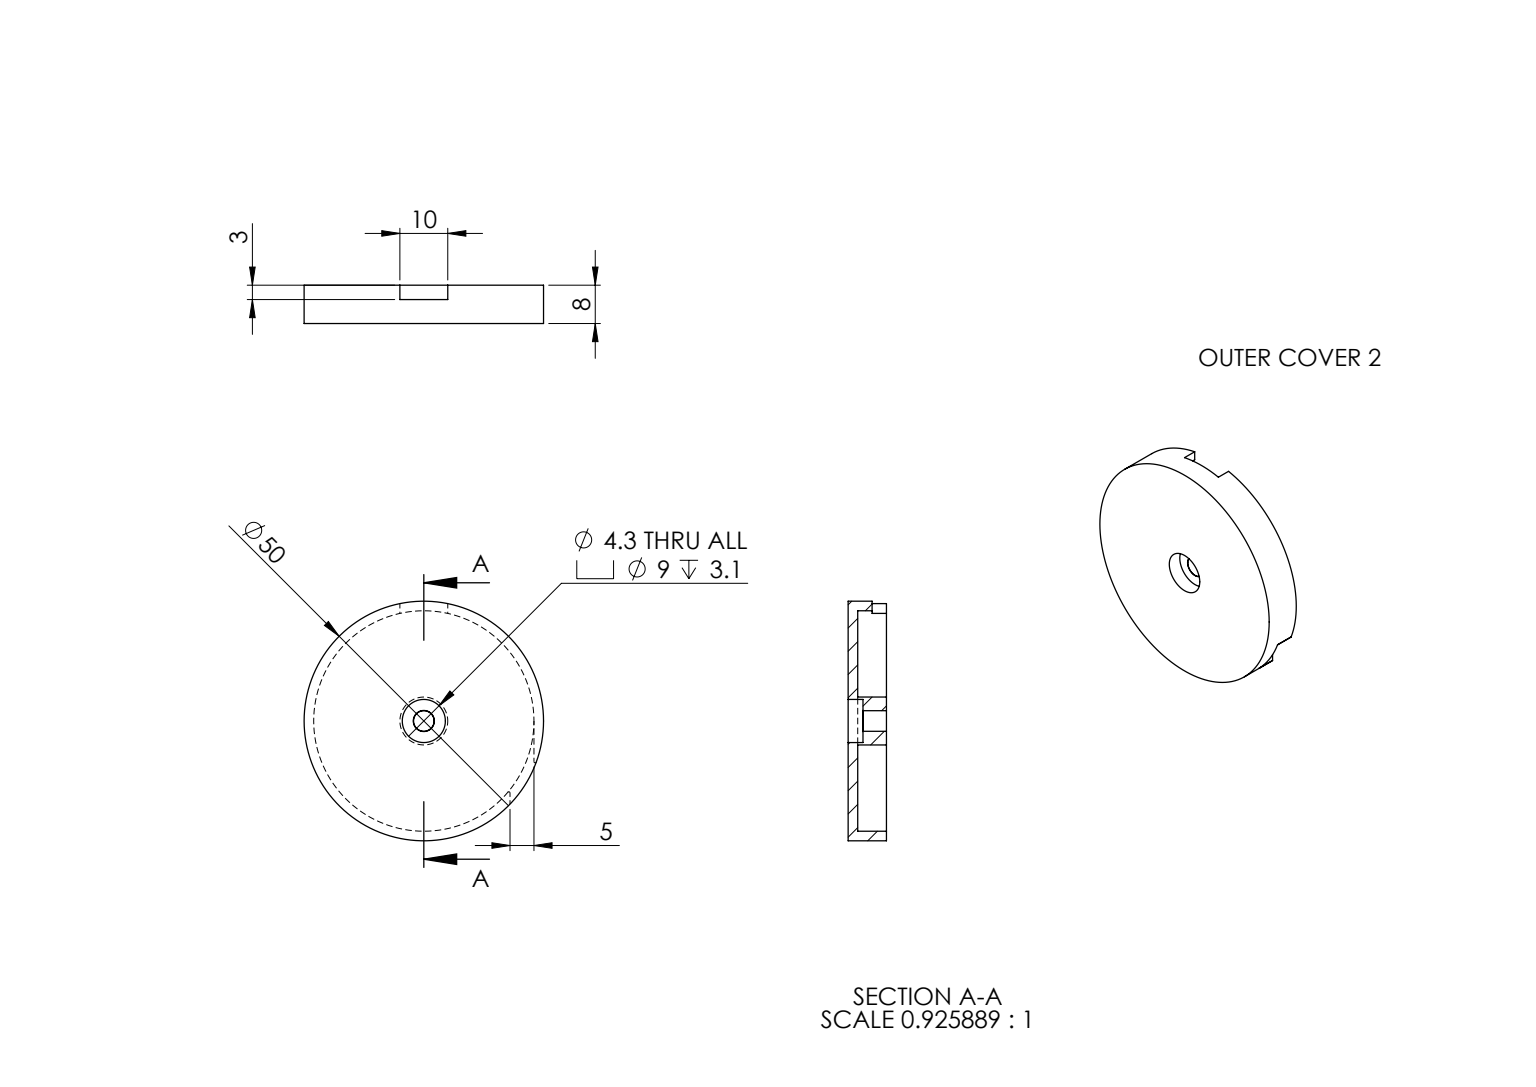
ISO-10303-21;
HEADER;
FILE_DESCRIPTION (('STEP AP214'),
    '1' );
FILE_NAME ('outer cover 2.step',
    '2026-10-23T14:45:25',
    ( '' ),
    ( '' ),
    'SwSTEP 2.0',
    'SolidWorks 2026',
    '' );
FILE_SCHEMA (( 'AUTOMOTIVE_DESIGN' ));
ENDSEC;

DATA;
#3=ORIENTED_EDGE ( 'NONE', *, *, #653, .T. ) ;
#4=EDGE_CURVE ( 'NONE', #1240, #2861, #1350, .T. ) ;
#28=FACE_OUTER_BOUND ( 'NONE', #3065, .T. ) ;
#29=CARTESIAN_POINT ( 'NONE',  ( -25.00000000000000000, 0.000000000000000000, -8.000000000000000000 ) ) ;
#36=VERTEX_POINT ( 'NONE', #2452 ) ;
#37=ORIENTED_EDGE ( 'NONE', *, *, #2017, .F. ) ;
#43=CIRCLE ( 'NONE', #2159, 23.00000000000000000 ) ;
#44=ORIENTED_EDGE ( 'NONE', *, *, #3966, .F. ) ;
#53=DIRECTION ( 'NONE',  ( -0.000000000000000000, -0.000000000000000000, -1.000000000000000000 ) ) ;
#56=CARTESIAN_POINT ( 'NONE',  ( 2.199999999999999289, 0.000000000000000000, -3.300000000000000266 ) ) ;
#58=EDGE_LOOP ( 'NONE', ( #1044, #3800, #158, #292 ) ) ;
#68=AXIS2_PLACEMENT_3D ( 'NONE', #3117, #2273, #3510 ) ;
#82=CARTESIAN_POINT ( 'NONE',  ( -2.149999999999997691, 2.632990618166807263E-16, -8.000000000000000000 ) ) ;
#85=DIRECTION ( 'NONE',  ( 0.000000000000000000, 0.000000000000000000, 1.000000000000000000 ) ) ;
#86=FACE_OUTER_BOUND ( 'NONE', #1906, .T. ) ;
#110=DIRECTION ( 'NONE',  ( -1.000000000000000000, 0.000000000000000000, 0.000000000000000000 ) ) ;
#118=VERTEX_POINT ( 'NONE', #3747 ) ;
#127=CIRCLE ( 'NONE', #405, 23.00000000000000000 ) ;
#130=AXIS2_PLACEMENT_3D ( 'NONE', #3700, #1115, #2554 ) ;
#146=DIRECTION ( 'NONE',  ( 1.000000000000000000, 0.000000000000000000, 0.000000000000000000 ) ) ;
#154=ADVANCED_FACE ( 'NONE', ( #5473 ), #2392, .F. ) ;
#158=ORIENTED_EDGE ( 'NONE', *, *, #190, .T. ) ;
#161=DIRECTION ( 'NONE',  ( -4.364351673553916694E-15, 1.000000000000000000, 0.000000000000000000 ) ) ;
#174=DIRECTION ( 'NONE',  ( 1.000000000000000000, 0.000000000000000000, 0.000000000000000000 ) ) ;
#190=EDGE_CURVE ( 'NONE', #442, #1012, #3278, .T. ) ;
#194=CARTESIAN_POINT ( 'NONE',  ( -25.00000000000000000, 0.000000000000000000, -8.000000000000000000 ) ) ;
#202=CARTESIAN_POINT ( 'NONE',  ( 25.00000000000000000, -3.061616997868383043E-15, -8.000000000000000000 ) ) ;
#204=ORIENTED_EDGE ( 'NONE', *, *, #5079, .F. ) ;
#207=DIRECTION ( 'NONE',  ( 1.000000000000000000, 0.000000000000000000, 0.000000000000000000 ) ) ;
#222=AXIS2_PLACEMENT_3D ( 'NONE', #3534, #53, #4345 ) ;
#225=( NAMED_UNIT ( * ) PLANE_ANGLE_UNIT ( ) SI_UNIT ( $, .RADIAN. ) );
#231=CARTESIAN_POINT ( 'NONE',  ( 0.000000000000000000, 0.000000000000000000, -3.106350832689629637 ) ) ;
#232=ORIENTED_EDGE ( 'NONE', *, *, #2358, .F. ) ;
#233=CIRCLE ( 'NONE', #3913, 2.149999999999997691 ) ;
#235=CARTESIAN_POINT ( 'NONE',  ( 0.000000000000000000, 0.000000000000000000, -8.000000000000000000 ) ) ;
#238=DIRECTION ( 'NONE',  ( -0.000000000000000000, -0.000000000000000000, -1.000000000000000000 ) ) ;
#239=ORIENTED_EDGE ( 'NONE', *, *, #2358, .T. ) ;
#247=VERTEX_POINT ( 'NONE', #3664 ) ;
#254=ORIENTED_EDGE ( 'NONE', *, *, #1540, .F. ) ;
#283=CARTESIAN_POINT ( 'NONE',  ( 0.000000000000000000, 0.000000000000000000, 0.000000000000000000 ) ) ;
#284=CARTESIAN_POINT ( 'NONE',  ( -5.000000000000000000, 0.000000000000000000, -2.000000000000000000 ) ) ;
#285=DIRECTION ( 'NONE',  ( -0.000000000000000000, -0.000000000000000000, 1.000000000000000000 ) ) ;
#287=CARTESIAN_POINT ( 'NONE',  ( 0.000000000000000000, 0.000000000000000000, -8.000000000000000000 ) ) ;
#292=ORIENTED_EDGE ( 'NONE', *, *, #2127, .F. ) ;
#298=PRODUCT_DEFINITION_FORMATION_WITH_SPECIFIED_SOURCE ( 'ANY', '', #4227, .NOT_KNOWN. ) ;
#313=DIRECTION ( 'NONE',  ( 0.000000000000000000, 0.000000000000000000, -1.000000000000000000 ) ) ;
#314=( LENGTH_UNIT ( ) NAMED_UNIT ( * ) SI_UNIT ( .MILLI., .METRE. ) );
#325=ORIENTED_EDGE ( 'NONE', *, *, #4902, .F. ) ;
#334=CIRCLE ( 'NONE', #715, 2.149999999999997691 ) ;
#342=CIRCLE ( 'NONE', #3844, 5.000000000000000000 ) ;
#347=CARTESIAN_POINT ( 'NONE',  ( 2.149999999999997691, 0.000000000000000000, -8.000000000000000000 ) ) ;
#352=EDGE_CURVE ( 'NONE', #3586, #36, #4839, .T. ) ;
#353=CARTESIAN_POINT ( 'NONE',  ( 23.00000000000000000, -2.816687638038912352E-15, -8.000000000000000000 ) ) ;
#354=VERTEX_POINT ( 'NONE', #2939 ) ;
#355=DIRECTION ( 'NONE',  ( -0.000000000000000000, -0.000000000000000000, 1.000000000000000000 ) ) ;
#370=FACE_OUTER_BOUND ( 'NONE', #4591, .T. ) ;
#379=ORIENTED_EDGE ( 'NONE', *, *, #1622, .F. ) ;
#387=ORIENTED_EDGE ( 'NONE', *, *, #3947, .T. ) ;
#401=CIRCLE ( 'NONE', #1231, 25.00000000000000000 ) ;
#403=VERTEX_POINT ( 'NONE', #4665 ) ;
#405=AXIS2_PLACEMENT_3D ( 'NONE', #490, #1846, #5415 ) ;
#410=CARTESIAN_POINT ( 'NONE',  ( 17.99999999999999289, -15.01665741768121443, -4.000000000000000000 ) ) ;
#412=EDGE_CURVE ( 'NONE', #4755, #1305, #3551, .T. ) ;
#418=DIRECTION ( 'NONE',  ( -0.000000000000000000, -0.000000000000000000, 1.000000000000000000 ) ) ;
#429=EDGE_CURVE ( 'NONE', #1326, #5392, #2179, .T. ) ;
#432=DIRECTION ( 'NONE',  ( 1.000000000000000000, 4.364351673553916694E-15, 0.000000000000000000 ) ) ;
#434=PLANE ( 'NONE',  #1688 ) ;
#437=LINE ( 'NONE', #5272, #4474 ) ;
#442=VERTEX_POINT ( 'NONE', #2044 ) ;
#447=DIRECTION ( 'NONE',  ( 1.000000000000000000, 0.000000000000000000, 0.000000000000000000 ) ) ;
#449=ORIENTED_EDGE ( 'NONE', *, *, #2127, .T. ) ;
#463=CARTESIAN_POINT ( 'NONE',  ( -5.000000000000076383, 22.44994432064363110, -8.000000000000000000 ) ) ;
#480=CARTESIAN_POINT ( 'NONE',  ( 5.000000000000000000, -6.123233995736766282E-16, -8.000000000000000000 ) ) ;
#485=ORIENTED_EDGE ( 'NONE', *, *, #2804, .F. ) ;
#488=ADVANCED_FACE ( 'NONE', ( #1241, #3003 ), #4748, .T. ) ;
#490=CARTESIAN_POINT ( 'NONE',  ( 0.000000000000000000, 0.000000000000000000, -4.000000000000000000 ) ) ;
#505=VECTOR ( 'NONE', #782, 1000.000000000000000 ) ;
#519=CARTESIAN_POINT ( 'NONE',  ( 0.000000000000000000, 0.000000000000000000, 0.000000000000000000 ) ) ;
#521=DIRECTION ( 'NONE',  ( 1.000000000000000000, 0.000000000000000000, 0.000000000000000000 ) ) ;
#529=VECTOR ( 'NONE', #2822, 1000.000000000000000 ) ;
#530=EDGE_CURVE ( 'NONE', #964, #1719, #3971, .T. ) ;
#533=VECTOR ( 'NONE', #2608, 1000.000000000000000 ) ;
#541=CARTESIAN_POINT ( 'NONE',  ( 4.999999999999914735, 24.49489742783179835, -8.000000000000000000 ) ) ;
#545=DIRECTION ( 'NONE',  ( -0.000000000000000000, -0.000000000000000000, 1.000000000000000000 ) ) ;
#547=CARTESIAN_POINT ( 'NONE',  ( 0.000000000000000000, 0.000000000000000000, -8.000000000000000000 ) ) ;
#559=EDGE_CURVE ( 'NONE', #5009, #2746, #334, .T. ) ;
#595=AXIS2_PLACEMENT_3D ( 'NONE', #235, #4212, #754 ) ;
#617=CARTESIAN_POINT ( 'NONE',  ( 0.000000000000000000, 0.000000000000000000, -2.000000000000000000 ) ) ;
#629=LINE ( 'NONE', #194, #3082 ) ;
#630=SURFACE_STYLE_FILL_AREA ( #1056 ) ;
#637=FACE_OUTER_BOUND ( 'NONE', #4150, .T. ) ;
#639=DIRECTION ( 'NONE',  ( 0.000000000000000000, 0.000000000000000000, -1.000000000000000000 ) ) ;
#640=ORIENTED_EDGE ( 'NONE', *, *, #4759, .T. ) ;
#653=EDGE_CURVE ( 'NONE', #2224, #1028, #888, .T. ) ;
#655=ORIENTED_EDGE ( 'NONE', *, *, #4575, .F. ) ;
#658=( LENGTH_UNIT ( ) NAMED_UNIT ( * ) SI_UNIT ( .MILLI., .METRE. ) );
#679=EDGE_CURVE ( 'NONE', #5392, #4001, #437, .T. ) ;
#684=PRODUCT_DEFINITION_SHAPE ( 'NONE', 'NONE',  #4858 ) ;
#685=CIRCLE ( 'NONE', #222, 0.2500000000000002220 ) ;
#697=DIRECTION ( 'NONE',  ( 1.000000000000000000, 0.000000000000000000, 0.000000000000000000 ) ) ;
#706=AXIS2_PLACEMENT_3D ( 'NONE', #231, #639, #3316 ) ;
#715=AXIS2_PLACEMENT_3D ( 'NONE', #547, #1756, #4837 ) ;
#726=VERTEX_POINT ( 'NONE', #4122 ) ;
#734=ORIENTED_EDGE ( 'NONE', *, *, #788, .F. ) ;
#749=DIRECTION ( 'NONE',  ( -1.000000000000000000, 0.000000000000000000, -0.000000000000000000 ) ) ;
#750=FACE_OUTER_BOUND ( 'NONE', #5246, .T. ) ;
#751=ORIENTED_EDGE ( 'NONE', *, *, #1982, .T. ) ;
#754=DIRECTION ( 'NONE',  ( 1.000000000000000000, 0.000000000000000000, 0.000000000000000000 ) ) ;
#777=AXIS2_PLACEMENT_3D ( 'NONE', #4406, #5273, #4868 ) ;
#782=DIRECTION ( 'NONE',  ( 0.000000000000000000, 0.000000000000000000, -1.000000000000000000 ) ) ;
#788=EDGE_CURVE ( 'NONE', #1305, #1719, #3740, .T. ) ;
#789=ORIENTED_EDGE ( 'NONE', *, *, #2529, .F. ) ;
#804=CARTESIAN_POINT ( 'NONE',  ( 0.000000000000000000, 0.000000000000000000, -8.000000000000000000 ) ) ;
#805=AXIS2_PLACEMENT_3D ( 'NONE', #2161, #2766, #5035 ) ;
#808=VECTOR ( 'NONE', #3588, 1000.000000000000000 ) ;
#810=DIRECTION ( 'NONE',  ( -0.000000000000000000, -0.000000000000000000, 1.000000000000000000 ) ) ;
#818=ORIENTED_EDGE ( 'NONE', *, *, #1286, .T. ) ;
#836=CARTESIAN_POINT ( 'NONE',  ( 23.00000000000000000, -2.168404344971008868E-16, -4.000000000000000000 ) ) ;
#840=LINE ( 'NONE', #2596, #1777 ) ;
#848=MECHANICAL_DESIGN_GEOMETRIC_PRESENTATION_REPRESENTATION('',(#4251),#2780);
#860=CARTESIAN_POINT ( 'NONE',  ( 23.00000000000000000, -2.168404344971008868E-16, -8.000000000000000000 ) ) ;
#862=CARTESIAN_POINT ( 'NONE',  ( 2.149999999999998579, 0.000000000000000000, 0.000000000000000000 ) ) ;
#864=DIRECTION ( 'NONE',  ( 1.000000000000000000, 0.000000000000000000, 0.000000000000000000 ) ) ;
#867=AXIS2_PLACEMENT_3D ( 'NONE', #4433, #2247, #5330 ) ;
#869=DIRECTION ( 'NONE',  ( -3.540989467475305966E-16, -1.000000000000000000, -0.000000000000000000 ) ) ;
#872=ORIENTED_EDGE ( 'NONE', *, *, #3851, .T. ) ;
#873=CIRCLE ( 'NONE', #595, 25.00000000000000000 ) ;
#878=FACE_OUTER_BOUND ( 'NONE', #5457, .T. ) ;
#882=AXIS2_PLACEMENT_3D ( 'NONE', #2501, #810, #3833 ) ;
#888=CIRCLE ( 'NONE', #3930, 4.500000000000000000 ) ;
#889=DIRECTION ( 'NONE',  ( -3.540989467475305966E-16, -1.000000000000000000, -0.000000000000000000 ) ) ;
#893=CARTESIAN_POINT ( 'NONE',  ( -23.00000000000000000, 0.000000000000000000, -8.000000000000000000 ) ) ;
#894=APPLICATION_CONTEXT ( 'automotive_design' ) ;
#896=DIRECTION ( 'NONE',  ( -4.364351673553916694E-15, 1.000000000000000000, 0.000000000000000000 ) ) ;
#901=ORIENTED_EDGE ( 'NONE', *, *, #5146, .T. ) ;
#920=CARTESIAN_POINT ( 'NONE',  ( 0.000000000000000000, 0.000000000000000000, -5.000000000000000000 ) ) ;
#921=DIRECTION ( 'NONE',  ( 1.000000000000000000, 0.000000000000000000, 0.000000000000000000 ) ) ;
#922=ORIENTED_EDGE ( 'NONE', *, *, #4867, .T. ) ;
#924=FACE_OUTER_BOUND ( 'NONE', #1877, .T. ) ;
#926=DIRECTION ( 'NONE',  ( -0.000000000000000000, -0.000000000000000000, 1.000000000000000000 ) ) ;
#929=ORIENTED_EDGE ( 'NONE', *, *, #5527, .F. ) ;
#948=DIRECTION ( 'NONE',  ( 0.000000000000000000, -1.000000000000000000, 0.000000000000000000 ) ) ;
#953=SHAPE_REPRESENTATION ( 'outer cover 2', ( #1336 ), #1859 ) ;
#964=VERTEX_POINT ( 'NONE', #4986 ) ;
#968=VECTOR ( 'NONE', #1615, 1000.000000000000000 ) ;
#971=ORIENTED_EDGE ( 'NONE', *, *, #1622, .T. ) ;
#974=DIRECTION ( 'NONE',  ( 0.000000000000000000, 0.000000000000000000, -1.000000000000000000 ) ) ;
#976=LINE ( 'NONE', #3168, #5554 ) ;
#978=PLANE ( 'NONE',  #1040 ) ;
#1009=FACE_BOUND ( 'NONE', #1425, .T. ) ;
#1011=CARTESIAN_POINT ( 'NONE',  ( 0.000000000000000000, 0.000000000000000000, -8.000000000000000000 ) ) ;
#1012=VERTEX_POINT ( 'NONE', #4674 ) ;
#1013=DIRECTION ( 'NONE',  ( -3.540989467475305966E-16, -1.000000000000000000, -0.000000000000000000 ) ) ;
#1028=VERTEX_POINT ( 'NONE', #2977 ) ;
#1033=DIRECTION ( 'NONE',  ( -3.540989467475305966E-16, -1.000000000000000000, -0.000000000000000000 ) ) ;
#1040=AXIS2_PLACEMENT_3D ( 'NONE', #2620, #432, #2736 ) ;
#1044=ORIENTED_EDGE ( 'NONE', *, *, #653, .F. ) ;
#1054=AXIS2_PLACEMENT_3D ( 'NONE', #2328, #1955, #1472 ) ;
#1056=FILL_AREA_STYLE ('',( #3198 ) ) ;
#1080=AXIS2_PLACEMENT_3D ( 'NONE', #5289, #3105, #5452 ) ;
#1090=DIRECTION ( 'NONE',  ( 1.000000000000000000, 0.000000000000000000, 0.000000000000000000 ) ) ;
#1106=ORIENTED_EDGE ( 'NONE', *, *, #4480, .T. ) ;
#1112=ORIENTED_EDGE ( 'NONE', *, *, #3851, .F. ) ;
#1115=DIRECTION ( 'NONE',  ( -0.000000000000000000, -0.000000000000000000, 1.000000000000000000 ) ) ;
#1121=FACE_OUTER_BOUND ( 'NONE', #1958, .T. ) ;
#1130=ORIENTED_EDGE ( 'NONE', *, *, #4867, .F. ) ;
#1143=FACE_OUTER_BOUND ( 'NONE', #1789, .T. ) ;
#1146=ORIENTED_EDGE ( 'NONE', *, *, #3983, .F. ) ;
#1150=CYLINDRICAL_SURFACE ( 'NONE', #4567, 25.00000000000000000 ) ;
#1154=CYLINDRICAL_SURFACE ( 'NONE', #882, 5.000000000000000000 ) ;
#1155=ORIENTED_EDGE ( 'NONE', *, *, #4164, .T. ) ;
#1165=FACE_OUTER_BOUND ( 'NONE', #5587, .T. ) ;
#1188=DIRECTION ( 'NONE',  ( -0.000000000000000000, -0.000000000000000000, -1.000000000000000000 ) ) ;
#1189=CARTESIAN_POINT ( 'NONE',  ( -4.500000000000000000, 5.510910596163088569E-16, -3.100000000000000533 ) ) ;
#1215=ORIENTED_EDGE ( 'NONE', *, *, #3973, .F. ) ;
#1221=ORIENTED_EDGE ( 'NONE', *, *, #3980, .F. ) ;
#1231=AXIS2_PLACEMENT_3D ( 'NONE', #5535, #4721, #2082 ) ;
#1240=VERTEX_POINT ( 'NONE', #3493 ) ;
#1241=FACE_BOUND ( 'NONE', #2539, .T. ) ;
#1243=AXIS2_PLACEMENT_3D ( 'NONE', #5613, #2971, #4485 ) ;
#1251=VERTEX_POINT ( 'NONE', #893 ) ;
#1256=CIRCLE ( 'NONE', #1987, 0.2000000000000000944 ) ;
#1271=LINE ( 'NONE', #836, #5014 ) ;
#1274=EDGE_CURVE ( 'NONE', #2861, #1240, #2182, .T. ) ;
#1275=DIRECTION ( 'NONE',  ( -1.000000000000000000, 0.000000000000000000, 0.000000000000000000 ) ) ;
#1280=CARTESIAN_POINT ( 'NONE',  ( -5.000000000000076383, 22.44994432064363110, -8.000000000000000000 ) ) ;
#1283=VERTEX_POINT ( 'NONE', #5298 ) ;
#1286=EDGE_CURVE ( 'NONE', #4444, #1251, #4750, .T. ) ;
#1300=LINE ( 'NONE', #5154, #4925 ) ;
#1303=CARTESIAN_POINT ( 'NONE',  ( 0.000000000000000000, 0.000000000000000000, -3.100000000000000533 ) ) ;
#1305=VERTEX_POINT ( 'NONE', #29 ) ;
#1326=VERTEX_POINT ( 'NONE', #2652 ) ;
#1335=DIRECTION ( 'NONE',  ( 1.000000000000000000, 0.000000000000000000, 0.000000000000000000 ) ) ;
#1336=AXIS2_PLACEMENT_3D ( 'NONE', #283, #2997, #5213 ) ;
#1339=VECTOR ( 'NONE', #4158, 1000.000000000000000 ) ;
#1350=CIRCLE ( 'NONE', #5207, 25.00000000000000000 ) ;
#1359=FACE_OUTER_BOUND ( 'NONE', #58, .T. ) ;
#1363=AXIS2_PLACEMENT_3D ( 'NONE', #3047, #2232, #4792 ) ;
#1368=EDGE_CURVE ( 'NONE', #4473, #118, #5491, .T. ) ;
#1385=DIRECTION ( 'NONE',  ( -0.000000000000000000, -0.000000000000000000, 1.000000000000000000 ) ) ;
#1388=CARTESIAN_POINT ( 'NONE',  ( 17.99999999999999289, -17.34935157289748631, -8.000000000000000000 ) ) ;
#1406=DIRECTION ( 'NONE',  ( -0.000000000000000000, -0.000000000000000000, 1.000000000000000000 ) ) ;
#1410=CARTESIAN_POINT ( 'NONE',  ( -2.149999999999998579, 2.632990618166807756E-16, 0.000000000000000000 ) ) ;
#1413=AXIS2_PLACEMENT_3D ( 'NONE', #3624, #3999, #2272 ) ;
#1416=ORIENTED_EDGE ( 'NONE', *, *, #5052, .T. ) ;
#1423=EDGE_CURVE ( 'NONE', #5009, #4159, #3539, .T. ) ;
#1425=EDGE_LOOP ( 'NONE', ( #1744, #4928 ) ) ;
#1429=CIRCLE ( 'NONE', #5468, 4.500000000000000000 ) ;
#1433=VECTOR ( 'NONE', #1967, 1000.000000000000000 ) ;
#1435=ADVANCED_FACE ( 'NONE', ( #1359 ), #4864, .F. ) ;
#1436=CARTESIAN_POINT ( 'NONE',  ( 0.000000000000000000, 0.000000000000000000, -5.000000000000000000 ) ) ;
#1438=AXIS2_PLACEMENT_3D ( 'NONE', #56, #948, #4057 ) ;
#1440=EDGE_LOOP ( 'NONE', ( #3729, #3554, #4497, #1761, #1130, #655 ) ) ;
#1442=CARTESIAN_POINT ( 'NONE',  ( -23.00000000000000000, 0.000000000000000000, -8.000000000000000000 ) ) ;
#1467=ADVANCED_FACE ( 'NONE', ( #86 ), #1841, .F. ) ;
#1472=DIRECTION ( 'NONE',  ( 1.000000000000000000, 0.000000000000000000, 0.000000000000000000 ) ) ;
#1479=LINE ( 'NONE', #3236, #1433 ) ;
#1507=CARTESIAN_POINT ( 'NONE',  ( -5.000000000000000000, 4.999999999999978684, -5.000000000000000000 ) ) ;
#1509=CIRCLE ( 'NONE', #777, 23.00000000000000000 ) ;
#1518=PRESENTATION_STYLE_ASSIGNMENT (( #5461 ) ) ;
#1525=CARTESIAN_POINT ( 'NONE',  ( 0.000000000000000000, 0.000000000000000000, -8.000000000000000000 ) ) ;
#1528=AXIS2_PLACEMENT_3D ( 'NONE', #2132, #2912, #2480 ) ;
#1531=ORIENTED_EDGE ( 'NONE', *, *, #4413, .F. ) ;
#1540=EDGE_CURVE ( 'NONE', #3849, #354, #342, .T. ) ;
#1541=ORIENTED_EDGE ( 'NONE', *, *, #3983, .T. ) ;
#1554=( LENGTH_UNIT ( ) NAMED_UNIT ( * ) SI_UNIT ( .MILLI., .METRE. ) );
#1556=VERTEX_POINT ( 'NONE', #1869 ) ;
#1563=DIRECTION ( 'NONE',  ( 1.000000000000000000, 0.000000000000000000, 0.000000000000000000 ) ) ;
#1577=FACE_OUTER_BOUND ( 'NONE', #5516, .T. ) ;
#1579=ORIENTED_EDGE ( 'NONE', *, *, #2603, .F. ) ;
#1592=ORIENTED_EDGE ( 'NONE', *, *, #530, .F. ) ;
#1604=AXIS2_PLACEMENT_3D ( 'NONE', #1750, #3479, #3652 ) ;
#1605=CYLINDRICAL_SURFACE ( 'NONE', #2246, 25.00000000000000000 ) ;
#1615=DIRECTION ( 'NONE',  ( -0.000000000000000000, -0.000000000000000000, 1.000000000000000000 ) ) ;
#1622=EDGE_CURVE ( 'NONE', #1251, #1556, #1925, .T. ) ;
#1631=AXIS2_PLACEMENT_3D ( 'NONE', #2021, #3289, #1563 ) ;
#1647=ORIENTED_EDGE ( 'NONE', *, *, #1995, .F. ) ;
#1651=ADVANCED_BREP_SHAPE_REPRESENTATION ( '', ( #2595, #1336 ), #1859 ) ;
#1654=DIRECTION ( 'NONE',  ( -0.000000000000000000, -0.000000000000000000, 1.000000000000000000 ) ) ;
#1671=CARTESIAN_POINT ( 'NONE',  ( -5.000000000000000000, 0.000000000000000000, -8.000000000000000000 ) ) ;
#1679=EDGE_LOOP ( 'NONE', ( #3362, #5619, #5333, #2493 ) ) ;
#1688=AXIS2_PLACEMENT_3D ( 'NONE', #2651, #85, #4800 ) ;
#1696=VECTOR ( 'NONE', #1406, 1000.000000000000000 ) ;
#1706=DIRECTION ( 'NONE',  ( 0.000000000000000000, 0.000000000000000000, -1.000000000000000000 ) ) ;
#1707=AXIS2_PLACEMENT_3D ( 'NONE', #3491, #355, #2109 ) ;
#1719=VERTEX_POINT ( 'NONE', #3282 ) ;
#1721=PLANE ( 'NONE',  #5033 ) ;
#1731=LINE ( 'NONE', #2999, #2262 ) ;
#1744=ORIENTED_EDGE ( 'NONE', *, *, #1866, .F. ) ;
#1745=DIRECTION ( 'NONE',  ( 1.000000000000000000, 4.364351673553916694E-15, 0.000000000000000000 ) ) ;
#1750=CARTESIAN_POINT ( 'NONE',  ( 0.000000000000000000, 0.000000000000000000, 0.000000000000000000 ) ) ;
#1754=DIRECTION ( 'NONE',  ( -0.000000000000000000, -0.000000000000000000, 1.000000000000000000 ) ) ;
#1756=DIRECTION ( 'NONE',  ( -0.000000000000000000, -0.000000000000000000, 1.000000000000000000 ) ) ;
#1761=ORIENTED_EDGE ( 'NONE', *, *, #4480, .F. ) ;
#1769=ORIENTED_EDGE ( 'NONE', *, *, #3650, .T. ) ;
#1771=LINE ( 'NONE', #3527, #533 ) ;
#1774=SHAPE_DEFINITION_REPRESENTATION ( #684, #953 ) ;
#1777=VECTOR ( 'NONE', #869, 1000.000000000000000 ) ;
#1781=CARTESIAN_POINT ( 'NONE',  ( 23.24999999999999645, -8.485281374238580199, -8.000000000000000000 ) ) ;
#1789=EDGE_LOOP ( 'NONE', ( #922, #4542, #3410, #4328 ) ) ;
#1790=AXIS2_PLACEMENT_3D ( 'NONE', #1436, #3194, #4944 ) ;
#1795=ADVANCED_FACE ( 'NONE', ( #3794 ), #1150, .T. ) ;
#1810=FACE_OUTER_BOUND ( 'NONE', #2083, .T. ) ;
#1812=CIRCLE ( 'NONE', #2462, 4.500000000000000888 ) ;
#1813=CYLINDRICAL_SURFACE ( 'NONE', #1413, 23.00000000000000000 ) ;
#1823=CARTESIAN_POINT ( 'NONE',  ( 0.000000000000000000, 0.000000000000000000, 0.000000000000000000 ) ) ;
#1833=PRODUCT_CONTEXT ( 'NONE', #1998, 'mechanical' ) ;
#1837=CARTESIAN_POINT ( 'NONE',  ( 22.99999999999999645, -8.485281374238580199, -8.000000000000000000 ) ) ;
#1841=CYLINDRICAL_SURFACE ( 'NONE', #805, 23.00000000000000000 ) ;
#1846=DIRECTION ( 'NONE',  ( -0.000000000000000000, -0.000000000000000000, -1.000000000000000000 ) ) ;
#1855=ORIENTED_EDGE ( 'NONE', *, *, #2354, .F. ) ;
#1857=CARTESIAN_POINT ( 'NONE',  ( -5.000000000000000000, 0.000000000000000000, -8.000000000000000000 ) ) ;
#1859=( GEOMETRIC_REPRESENTATION_CONTEXT ( 3 ) GLOBAL_UNCERTAINTY_ASSIGNED_CONTEXT ( ( #2115 ) ) GLOBAL_UNIT_ASSIGNED_CONTEXT ( ( #658, #225, #5030 ) ) REPRESENTATION_CONTEXT ( 'NONE', 'WORKASPACE' ) );
#1866=EDGE_CURVE ( 'NONE', #1012, #442, #1812, .T. ) ;
#1868=DIRECTION ( 'NONE',  ( -0.000000000000000000, -0.000000000000000000, -1.000000000000000000 ) ) ;
#1869=CARTESIAN_POINT ( 'NONE',  ( -23.00000000000000000, 0.000000000000000000, -2.000000000000000000 ) ) ;
#1870=VECTOR ( 'NONE', #3544, 1000.000000000000000 ) ;
#1874=FACE_OUTER_BOUND ( 'NONE', #2278, .T. ) ;
#1875=DIRECTION ( 'NONE',  ( -1.000000000000000000, 0.000000000000000000, 0.000000000000000000 ) ) ;
#1877=EDGE_LOOP ( 'NONE', ( #2752, #4571, #2770, #44 ) ) ;
#1883=AXIS2_PLACEMENT_3D ( 'NONE', #3941, #2586, #4886 ) ;
#1906=EDGE_LOOP ( 'NONE', ( #4564, #3540, #1647, #2028, #971, #2722 ) ) ;
#1925=LINE ( 'NONE', #1442, #529 ) ;
#1935=ADVANCED_FACE ( 'NONE', ( #4419 ), #1721, .F. ) ;
#1947=DIRECTION ( 'NONE',  ( -0.000000000000000000, -0.000000000000000000, 1.000000000000000000 ) ) ;
#1955=DIRECTION ( 'NONE',  ( -0.000000000000000000, -0.000000000000000000, 1.000000000000000000 ) ) ;
#1958=EDGE_LOOP ( 'NONE', ( #4056, #387, #2428, #1215 ) ) ;
#1960=LINE ( 'NONE', #541, #505 ) ;
#1967=DIRECTION ( 'NONE',  ( -0.000000000000000000, -0.000000000000000000, 1.000000000000000000 ) ) ;
#1979=CARTESIAN_POINT ( 'NONE',  ( 17.74999999999999289, -15.01665741768121443, -8.000000000000000000 ) ) ;
#1981=VECTOR ( 'NONE', #3298, 1000.000000000000000 ) ;
#1982=EDGE_CURVE ( 'NONE', #118, #4473, #4572, .T. ) ;
#1987=AXIS2_PLACEMENT_3D ( 'NONE', #4347, #4489, #3509 ) ;
#1989=AXIS2_PLACEMENT_3D ( 'NONE', #2163, #1188, #1275 ) ;
#1995=EDGE_CURVE ( 'NONE', #5065, #4764, #1771, .T. ) ;
#1998=APPLICATION_CONTEXT ( 'automotive_design' ) ;
#2001=CARTESIAN_POINT ( 'NONE',  ( 4.999999999999923617, 22.44994432064366308, -5.000000000000000000 ) ) ;
#2013=ORIENTED_EDGE ( 'NONE', *, *, #4, .T. ) ;
#2017=EDGE_CURVE ( 'NONE', #2140, #4992, #4026, .T. ) ;
#2021=CARTESIAN_POINT ( 'NONE',  ( 0.000000000000000000, 0.000000000000000000, 0.000000000000000000 ) ) ;
#2028=ORIENTED_EDGE ( 'NONE', *, *, #5146, .F. ) ;
#2032=EDGE_CURVE ( 'NONE', #403, #5536, #4075, .T. ) ;
#2043=ORIENTED_EDGE ( 'NONE', *, *, #530, .T. ) ;
#2044=CARTESIAN_POINT ( 'NONE',  ( -4.500000000000000888, 5.510910596163089556E-16, 0.000000000000000000 ) ) ;
#2050=ORIENTED_EDGE ( 'NONE', *, *, #2603, .T. ) ;
#2058=AXIS2_PLACEMENT_3D ( 'NONE', #2680, #4895, #1033 ) ;
#2068=AXIS2_PLACEMENT_3D ( 'NONE', #3708, #4178, #697 ) ;
#2078=DIRECTION ( 'NONE',  ( -0.000000000000000000, -0.000000000000000000, 1.000000000000000000 ) ) ;
#2082=DIRECTION ( 'NONE',  ( 1.000000000000000000, 0.000000000000000000, 0.000000000000000000 ) ) ;
#2083=EDGE_LOOP ( 'NONE', ( #2944, #734, #5367, #4678, #818, #901, #1855 ) ) ;
#2105=LINE ( 'NONE', #1837, #3908 ) ;
#2107=DIRECTION ( 'NONE',  ( 1.000000000000000000, 0.000000000000000000, 0.000000000000000000 ) ) ;
#2109=DIRECTION ( 'NONE',  ( 1.000000000000000000, 0.000000000000000000, 0.000000000000000000 ) ) ;
#2115=UNCERTAINTY_MEASURE_WITH_UNIT (LENGTH_MEASURE( 1.000000000000000082E-05 ), #658, 'distance_accuracy_value', 'NONE');
#2119=EDGE_LOOP ( 'NONE', ( #2510, #239, #3392, #1112 ) ) ;
#2125=DIRECTION ( 'NONE',  ( -1.000000000000000000, 0.000000000000000000, 0.000000000000000000 ) ) ;
#2127=EDGE_CURVE ( 'NONE', #1028, #1012, #2314, .T. ) ;
#2132=CARTESIAN_POINT ( 'NONE',  ( 0.000000000000000000, 0.000000000000000000, -8.000000000000000000 ) ) ;
#2140=VERTEX_POINT ( 'NONE', #1857 ) ;
#2159=AXIS2_PLACEMENT_3D ( 'NONE', #2408, #4540, #3197 ) ;
#2161=CARTESIAN_POINT ( 'NONE',  ( 0.000000000000000000, 0.000000000000000000, -8.000000000000000000 ) ) ;
#2163=CARTESIAN_POINT ( 'NONE',  ( 23.24999999999999645, -8.485281374238580199, -4.000000000000000000 ) ) ;
#2168=VERTEX_POINT ( 'NONE', #4938 ) ;
#2169=CARTESIAN_POINT ( 'NONE',  ( 0.000000000000000000, 0.000000000000000000, -8.000000000000000000 ) ) ;
#2175=AXIS2_PLACEMENT_3D ( 'NONE', #920, #1868, #110 ) ;
#2179=CIRCLE ( 'NONE', #2729, 23.00000000000000000 ) ;
#2182=CIRCLE ( 'NONE', #2915, 25.00000000000000000 ) ;
#2184=ORIENTED_EDGE ( 'NONE', *, *, #4565, .F. ) ;
#2187=PLANE ( 'NONE',  #1883 ) ;
#2193=DIRECTION ( 'NONE',  ( 0.000000000000000000, 0.000000000000000000, -1.000000000000000000 ) ) ;
#2198=ORIENTED_EDGE ( 'NONE', *, *, #3915, .F. ) ;
#2204=DIRECTION ( 'NONE',  ( 0.000000000000000000, 0.000000000000000000, -1.000000000000000000 ) ) ;
#2219=EDGE_LOOP ( 'NONE', ( #4311, #3579, #2918, #5649 ) ) ;
#2222=DIRECTION ( 'NONE',  ( -0.000000000000000000, -0.000000000000000000, 1.000000000000000000 ) ) ;
#2224=VERTEX_POINT ( 'NONE', #1189 ) ;
#2228=EDGE_CURVE ( 'NONE', #247, #4608, #873, .T. ) ;
#2232=DIRECTION ( 'NONE',  ( -0.000000000000000000, -0.000000000000000000, 1.000000000000000000 ) ) ;
#2242=LINE ( 'NONE', #862, #5205 ) ;
#2246=AXIS2_PLACEMENT_3D ( 'NONE', #3764, #4228, #4682 ) ;
#2247=DIRECTION ( 'NONE',  ( -0.000000000000000000, -0.000000000000000000, 1.000000000000000000 ) ) ;
#2248=PLANE ( 'NONE',  #2058 ) ;
#2255=AXIS2_PLACEMENT_3D ( 'NONE', #617, #5537, #3692 ) ;
#2262=VECTOR ( 'NONE', #313, 1000.000000000000000 ) ;
#2269=LINE ( 'NONE', #4453, #2615 ) ;
#2272=DIRECTION ( 'NONE',  ( -1.000000000000000000, 0.000000000000000000, 0.000000000000000000 ) ) ;
#2273=DIRECTION ( 'NONE',  ( -0.000000000000000000, -0.000000000000000000, 1.000000000000000000 ) ) ;
#2278=EDGE_LOOP ( 'NONE', ( #2198, #3250, #5233, #4878 ) ) ;
#2294=( NAMED_UNIT ( * ) SI_UNIT ( $, .STERADIAN. ) SOLID_ANGLE_UNIT ( ) );
#2298=DIRECTION ( 'NONE',  ( -0.000000000000000000, -0.000000000000000000, 1.000000000000000000 ) ) ;
#2300=EDGE_CURVE ( 'NONE', #1028, #2224, #1429, .T. ) ;
#2314=LINE ( 'NONE', #3695, #808 ) ;
#2328=CARTESIAN_POINT ( 'NONE',  ( 0.000000000000000000, 0.000000000000000000, -3.300000000000000266 ) ) ;
#2354=EDGE_CURVE ( 'NONE', #4137, #5065, #5382, .T. ) ;
#2358=EDGE_CURVE ( 'NONE', #2168, #4001, #1960, .T. ) ;
#2366=AXIS2_PLACEMENT_3D ( 'NONE', #519, #2677, #921 ) ;
#2371=CARTESIAN_POINT ( 'NONE',  ( 5.000000000000000000, 5.000000000000022204, -5.000000000000000000 ) ) ;
#2392=PLANE ( 'NONE',  #5300 ) ;
#2393=DIRECTION ( 'NONE',  ( -0.000000000000000000, -0.000000000000000000, 1.000000000000000000 ) ) ;
#2408=CARTESIAN_POINT ( 'NONE',  ( 0.000000000000000000, 0.000000000000000000, -8.000000000000000000 ) ) ;
#2417=CARTESIAN_POINT ( 'NONE',  ( 23.48484848484848442, -8.570991287109677614, -4.000000000000000000 ) ) ;
#2418=ORIENTED_EDGE ( 'NONE', *, *, #5527, .T. ) ;
#2419=CARTESIAN_POINT ( 'NONE',  ( 18.00000000000000000, 1.553654299240552096E-15, 16.41957833606399930 ) ) ;
#2422=AXIS2_PLACEMENT_3D ( 'NONE', #4327, #3514, #2107 ) ;
#2428=ORIENTED_EDGE ( 'NONE', *, *, #2544, .T. ) ;
#2435=ORIENTED_EDGE ( 'NONE', *, *, #5235, .T. ) ;
#2450=FACE_OUTER_BOUND ( 'NONE', #2890, .T. ) ;
#2452=CARTESIAN_POINT ( 'NONE',  ( 22.99999999999999645, -8.485281374238580199, -4.000000000000000000 ) ) ;
#2460=LINE ( 'NONE', #5108, #1981 ) ;
#2462=AXIS2_PLACEMENT_3D ( 'NONE', #3769, #5206, #2960 ) ;
#2467=EDGE_LOOP ( 'NONE', ( #3465, #1416, #5107, #3219, #3354, #1592, #3519, #2569 ) ) ;
#2478=CARTESIAN_POINT ( 'NONE',  ( 5.000000000000000000, -6.123233995736766282E-16, -8.000000000000000000 ) ) ;
#2479=ORIENTED_EDGE ( 'NONE', *, *, #2700, .T. ) ;
#2480=DIRECTION ( 'NONE',  ( 1.000000000000000000, 0.000000000000000000, 0.000000000000000000 ) ) ;
#2493=ORIENTED_EDGE ( 'NONE', *, *, #2950, .T. ) ;
#2500=DIRECTION ( 'NONE',  ( -3.540989467475305966E-16, -1.000000000000000000, -0.000000000000000000 ) ) ;
#2501=CARTESIAN_POINT ( 'NONE',  ( 0.000000000000000000, 0.000000000000000000, -8.000000000000000000 ) ) ;
#2502=ORIENTED_EDGE ( 'NONE', *, *, #4759, .F. ) ;
#2510=ORIENTED_EDGE ( 'NONE', *, *, #2804, .T. ) ;
#2529=EDGE_CURVE ( 'NONE', #3158, #4137, #5642, .T. ) ;
#2535=EDGE_CURVE ( 'NONE', #36, #726, #2105, .T. ) ;
#2537=CLOSED_SHELL ( 'NONE', ( #5675, #1435, #3259, #3997, #1795, #5533, #5063, #5017, #5428, #4827, #5266, #1467, #2995, #2663, #488, #154, #4509, #4025, #1935, #4146, #2588, #3195, #5328, #3909, #3154, #3661 ) ) ;
#2539=EDGE_LOOP ( 'NONE', ( #4970, #3860 ) ) ;
#2544=EDGE_CURVE ( 'NONE', #4159, #4295, #5196, .T. ) ;
#2554=DIRECTION ( 'NONE',  ( 1.000000000000000000, 0.000000000000000000, 0.000000000000000000 ) ) ;
#2565=CARTESIAN_POINT ( 'NONE',  ( 17.99999999999999289, -15.01665741768121443, -8.000000000000000000 ) ) ;
#2568=DIRECTION ( 'NONE',  ( -0.000000000000000000, -0.000000000000000000, 1.000000000000000000 ) ) ;
#2569=ORIENTED_EDGE ( 'NONE', *, *, #2896, .F. ) ;
#2586=DIRECTION ( 'NONE',  ( 0.000000000000000000, 0.000000000000000000, -1.000000000000000000 ) ) ;
#2588=ADVANCED_FACE ( 'NONE', ( #5378 ), #4425, .F. ) ;
#2593=COLOUR_RGB ( '',0.8941176470588234615, 0.8941176470588234615, 0.8941176470588234615 ) ;
#2595=MANIFOLD_SOLID_BREP ( '<outer cover 1>-<Fillet1>', #2537 ) ;
#2596=CARTESIAN_POINT ( 'NONE',  ( 18.00000000000000000, 1.553654299240552096E-15, -4.000000000000000000 ) ) ;
#2603=EDGE_CURVE ( 'NONE', #4992, #354, #5217, .T. ) ;
#2607=CIRCLE ( 'NONE', #2422, 23.00000000000000000 ) ;
#2608=DIRECTION ( 'NONE',  ( -0.000000000000000000, -0.000000000000000000, 1.000000000000000000 ) ) ;
#2610=CIRCLE ( 'NONE', #2892, 23.00000000000000000 ) ;
#2615=VECTOR ( 'NONE', #5323, 1000.000000000000000 ) ;
#2620=CARTESIAN_POINT ( 'NONE',  ( -5.000000000000000000, 4.999999999999978684, -5.000000000000000000 ) ) ;
#2631=ORIENTED_EDGE ( 'NONE', *, *, #4413, .T. ) ;
#2633=ORIENTED_EDGE ( 'NONE', *, *, #3973, .T. ) ;
#2636=AXIS2_PLACEMENT_3D ( 'NONE', #2797, #4547, #3685 ) ;
#2637=PLANE ( 'NONE',  #5644 ) ;
#2651=CARTESIAN_POINT ( 'NONE',  ( 0.000000000000000000, 0.000000000000000000, -4.000000000000000000 ) ) ;
#2652=CARTESIAN_POINT ( 'NONE',  ( 23.00000000000000000, -2.168404344971008868E-16, -8.000000000000000000 ) ) ;
#2653=ORIENTED_EDGE ( 'NONE', *, *, #2300, .T. ) ;
#2663=ADVANCED_FACE ( 'NONE', ( #750 ), #1154, .T. ) ;
#2674=LINE ( 'NONE', #860, #3441 ) ;
#2677=DIRECTION ( 'NONE',  ( -0.000000000000000000, -0.000000000000000000, 1.000000000000000000 ) ) ;
#2679=CYLINDRICAL_SURFACE ( 'NONE', #867, 2.149999999999998579 ) ;
#2680=CARTESIAN_POINT ( 'NONE',  ( 23.00000000000000000, -2.168404344971008868E-16, 16.41957833606399930 ) ) ;
#2700=EDGE_CURVE ( 'NONE', #2140, #3849, #5610, .T. ) ;
#2709=CIRCLE ( 'NONE', #130, 5.000000000000000000 ) ;
#2722=ORIENTED_EDGE ( 'NONE', *, *, #4565, .T. ) ;
#2726=CIRCLE ( 'NONE', #1438, 0.2000000000000000944 ) ;
#2729=AXIS2_PLACEMENT_3D ( 'NONE', #287, #2078, #3835 ) ;
#2736=DIRECTION ( 'NONE',  ( -4.364351673553916694E-15, 1.000000000000000000, 0.000000000000000000 ) ) ;
#2746=VERTEX_POINT ( 'NONE', #347 ) ;
#2752=ORIENTED_EDGE ( 'NONE', *, *, #559, .F. ) ;
#2762=SHAPE_REPRESENTATION_RELATIONSHIP ( 'NONE' , 'NONE' ,  #953, #1651 ) ;
#2766=DIRECTION ( 'NONE',  ( -0.000000000000000000, -0.000000000000000000, 1.000000000000000000 ) ) ;
#2770=ORIENTED_EDGE ( 'NONE', *, *, #3650, .F. ) ;
#2780=( GEOMETRIC_REPRESENTATION_CONTEXT ( 3 ) GLOBAL_UNCERTAINTY_ASSIGNED_CONTEXT ( ( #3898 ) ) GLOBAL_UNIT_ASSIGNED_CONTEXT ( ( #1554, #3653, #2294 ) ) REPRESENTATION_CONTEXT ( 'NONE', 'WORKASPACE' ) );
#2784=CARTESIAN_POINT ( 'NONE',  ( -4.500000000000000888, 5.510910596163089556E-16, 0.000000000000000000 ) ) ;
#2797=CARTESIAN_POINT ( 'NONE',  ( 0.000000000000000000, 0.000000000000000000, -3.300000000000000266 ) ) ;
#2799=DIRECTION ( 'NONE',  ( -1.000000000000000000, 3.540989467475305966E-16, 0.000000000000000000 ) ) ;
#2804=EDGE_CURVE ( 'NONE', #2920, #2168, #4984, .T. ) ;
#2822=DIRECTION ( 'NONE',  ( -0.000000000000000000, -0.000000000000000000, 1.000000000000000000 ) ) ;
#2861=VERTEX_POINT ( 'NONE', #4131 ) ;
#2890=EDGE_LOOP ( 'NONE', ( #3511, #751, #2633, #1769 ) ) ;
#2892=AXIS2_PLACEMENT_3D ( 'NONE', #4521, #926, #146 ) ;
#2896=EDGE_CURVE ( 'NONE', #247, #3586, #1479, .T. ) ;
#2898=EDGE_LOOP ( 'NONE', ( #1106, #2043, #204, #789 ) ) ;
#2910=( NAMED_UNIT ( * ) SI_UNIT ( $, .STERADIAN. ) SOLID_ANGLE_UNIT ( ) );
#2911=ORIENTED_EDGE ( 'NONE', *, *, #2228, .F. ) ;
#2912=DIRECTION ( 'NONE',  ( -0.000000000000000000, -0.000000000000000000, 1.000000000000000000 ) ) ;
#2915=AXIS2_PLACEMENT_3D ( 'NONE', #3917, #1754, #5671 ) ;
#2918=ORIENTED_EDGE ( 'NONE', *, *, #3966, .T. ) ;
#2920=VERTEX_POINT ( 'NONE', #2001 ) ;
#2929=CARTESIAN_POINT ( 'NONE',  ( 4.999999999999923617, 22.44994432064366308, -8.000000000000000000 ) ) ;
#2936=CARTESIAN_POINT ( 'NONE',  ( 2.149999999999999467, 0.000000000000000000, -3.100000000000000533 ) ) ;
#2939=CARTESIAN_POINT ( 'NONE',  ( 5.000000000000000000, -6.123233995736766282E-16, -2.000000000000000000 ) ) ;
#2943=CARTESIAN_POINT ( 'NONE',  ( 0.000000000000000000, 0.000000000000000000, -4.000000000000000000 ) ) ;
#2944=ORIENTED_EDGE ( 'NONE', *, *, #5079, .T. ) ;
#2945=CYLINDRICAL_SURFACE ( 'NONE', #1707, 4.500000000000000888 ) ;
#2950=EDGE_CURVE ( 'NONE', #4444, #4755, #2460, .T. ) ;
#2960=DIRECTION ( 'NONE',  ( 1.000000000000000000, 0.000000000000000000, 0.000000000000000000 ) ) ;
#2971=DIRECTION ( 'NONE',  ( 0.000000000000000000, 0.000000000000000000, -1.000000000000000000 ) ) ;
#2977=CARTESIAN_POINT ( 'NONE',  ( 4.500000000000000000, 0.000000000000000000, -3.100000000000000533 ) ) ;
#2980=AXIS2_PLACEMENT_3D ( 'NONE', #2943, #238, #4695 ) ;
#2992=AXIS2_PLACEMENT_3D ( 'NONE', #4583, #2393, #207 ) ;
#2995=ADVANCED_FACE ( 'NONE', ( #3325, #1165 ), #3782, .T. ) ;
#2997=DIRECTION ( 'NONE',  ( 0.000000000000000000, 0.000000000000000000, 1.000000000000000000 ) ) ;
#2999=CARTESIAN_POINT ( 'NONE',  ( 4.999999999999923617, 22.44994432064366308, -8.000000000000000000 ) ) ;
#3002=TOROIDAL_SURFACE ( 'NONE', #2636, 2.199999999999999289, 0.2000000000000000111 ) ;
#3003=FACE_OUTER_BOUND ( 'NONE', #3402, .T. ) ;
#3007=LINE ( 'NONE', #463, #1870 ) ;
#3047=CARTESIAN_POINT ( 'NONE',  ( 0.000000000000000000, 0.000000000000000000, -3.100000000000000533 ) ) ;
#3056=FACE_OUTER_BOUND ( 'NONE', #1679, .T. ) ;
#3059=DIRECTION ( 'NONE',  ( -0.000000000000000000, -0.000000000000000000, 1.000000000000000000 ) ) ;
#3061=DIRECTION ( 'NONE',  ( -0.000000000000000000, -0.000000000000000000, 1.000000000000000000 ) ) ;
#3065=EDGE_LOOP ( 'NONE', ( #4784, #4891, #2631, #379, #3258, #4716, #2418, #872, #3280 ) ) ;
#3075=CIRCLE ( 'NONE', #5456, 0.2500000000000002220 ) ;
#3082=VECTOR ( 'NONE', #1947, 1000.000000000000000 ) ;
#3085=TOROIDAL_SURFACE ( 'NONE', #1054, 2.199999999999999289, 0.2000000000000000111 ) ;
#3090=EDGE_CURVE ( 'NONE', #2746, #5009, #233, .T. ) ;
#3099=AXIS2_PLACEMENT_3D ( 'NONE', #3888, #5641, #521 ) ;
#3105=DIRECTION ( 'NONE',  ( -0.000000000000000000, -0.000000000000000000, 1.000000000000000000 ) ) ;
#3111=DIRECTION ( 'NONE',  ( 0.000000000000000000, 0.000000000000000000, -1.000000000000000000 ) ) ;
#3117=CARTESIAN_POINT ( 'NONE',  ( 0.000000000000000000, 0.000000000000000000, -8.000000000000000000 ) ) ;
#3122=FACE_OUTER_BOUND ( 'NONE', #3789, .T. ) ;
#3129=ORIENTED_EDGE ( 'NONE', *, *, #3980, .T. ) ;
#3131=CARTESIAN_POINT ( 'NONE',  ( 5.000000000000000000, 5.000000000000022204, -5.000000000000000000 ) ) ;
#3154=ADVANCED_FACE ( 'NONE', ( #4356 ), #2945, .F. ) ;
#3158=VERTEX_POINT ( 'NONE', #410 ) ;
#3167=CIRCLE ( 'NONE', #2980, 25.00000000000000000 ) ;
#3168=CARTESIAN_POINT ( 'NONE',  ( 18.00000000000000000, 1.553654299240552096E-15, -8.000000000000000000 ) ) ;
#3170=DIRECTION ( 'NONE',  ( 1.000000000000000000, 0.000000000000000000, 0.000000000000000000 ) ) ;
#3194=DIRECTION ( 'NONE',  ( 0.000000000000000000, 0.000000000000000000, 1.000000000000000000 ) ) ;
#3195=ADVANCED_FACE ( 'NONE', ( #3842 ), #5594, .T. ) ;
#3197=DIRECTION ( 'NONE',  ( 1.000000000000000000, 0.000000000000000000, 0.000000000000000000 ) ) ;
#3198=FILL_AREA_STYLE_COLOUR ( '', #2593 ) ;
#3219=ORIENTED_EDGE ( 'NONE', *, *, #5235, .F. ) ;
#3228=PLANE ( 'NONE',  #2068 ) ;
#3236=CARTESIAN_POINT ( 'NONE',  ( 23.48484848484848442, -8.570991287109677614, -8.000000000000000000 ) ) ;
#3250=ORIENTED_EDGE ( 'NONE', *, *, #4431, .T. ) ;
#3258=ORIENTED_EDGE ( 'NONE', *, *, #1286, .F. ) ;
#3259=ADVANCED_FACE ( 'NONE', ( #3122 ), #4954, .T. ) ;
#3266=STYLED_ITEM('',(#5709),#2595);
#3278=CIRCLE ( 'NONE', #1631, 4.500000000000000888 ) ;
#3280=ORIENTED_EDGE ( 'NONE', *, *, #429, .F. ) ;
#3282=CARTESIAN_POINT ( 'NONE',  ( 17.99999999999999289, -17.34935157289748631, -8.000000000000000000 ) ) ;
#3289=DIRECTION ( 'NONE',  ( -0.000000000000000000, -0.000000000000000000, 1.000000000000000000 ) ) ;
#3298=DIRECTION ( 'NONE',  ( -4.364351673553916694E-15, 1.000000000000000000, 0.000000000000000000 ) ) ;
#3307=DIRECTION ( 'NONE',  ( -1.000000000000000000, 0.000000000000000000, 0.000000000000000000 ) ) ;
#3316=DIRECTION ( 'NONE',  ( -1.000000000000000000, 0.000000000000000000, 0.000000000000000000 ) ) ;
#3325=FACE_BOUND ( 'NONE', #3385, .T. ) ;
#3332=ORIENTED_EDGE ( 'NONE', *, *, #412, .T. ) ;
#3345=EDGE_LOOP ( 'NONE', ( #4975, #5250, #1541, #5450 ) ) ;
#3347=DIRECTION ( 'NONE',  ( 1.000000000000000000, 0.000000000000000000, 0.000000000000000000 ) ) ;
#3349=CIRCLE ( 'NONE', #4633, 5.000000000000000000 ) ;
#3354=ORIENTED_EDGE ( 'NONE', *, *, #788, .T. ) ;
#3362=ORIENTED_EDGE ( 'NONE', *, *, #3752, .F. ) ;
#3365=DIRECTION ( 'NONE',  ( -0.000000000000000000, -0.000000000000000000, 1.000000000000000000 ) ) ;
#3385=EDGE_LOOP ( 'NONE', ( #3524, #640 ) ) ;
#3392=ORIENTED_EDGE ( 'NONE', *, *, #679, .F. ) ;
#3397=DIRECTION ( 'NONE',  ( -0.000000000000000000, -0.000000000000000000, 1.000000000000000000 ) ) ;
#3402=EDGE_LOOP ( 'NONE', ( #37, #3641 ) ) ;
#3410=ORIENTED_EDGE ( 'NONE', *, *, #2354, .T. ) ;
#3431=LINE ( 'NONE', #353, #5274 ) ;
#3433=DIRECTION ( 'NONE',  ( -0.000000000000000000, -0.000000000000000000, 1.000000000000000000 ) ) ;
#3441=VECTOR ( 'NONE', #889, 1000.000000000000000 ) ;
#3449=AXIS2_PLACEMENT_3D ( 'NONE', #1011, #2222, #1875 ) ;
#3452=PLANE ( 'NONE',  #3919 ) ;
#3465=ORIENTED_EDGE ( 'NONE', *, *, #2228, .T. ) ;
#3479=DIRECTION ( 'NONE',  ( -0.000000000000000000, -0.000000000000000000, 1.000000000000000000 ) ) ;
#3491=CARTESIAN_POINT ( 'NONE',  ( 0.000000000000000000, 0.000000000000000000, 0.000000000000000000 ) ) ;
#3493=CARTESIAN_POINT ( 'NONE',  ( 25.00000000000000000, -3.061616997868383043E-15, 0.000000000000000000 ) ) ;
#3509=DIRECTION ( 'NONE',  ( -1.000000000000000000, 1.224646799147353207E-16, 0.000000000000000000 ) ) ;
#3510=DIRECTION ( 'NONE',  ( 1.000000000000000000, 0.000000000000000000, 0.000000000000000000 ) ) ;
#3511=ORIENTED_EDGE ( 'NONE', *, *, #3947, .F. ) ;
#3514=DIRECTION ( 'NONE',  ( -0.000000000000000000, -0.000000000000000000, 1.000000000000000000 ) ) ;
#3519=ORIENTED_EDGE ( 'NONE', *, *, #4176, .F. ) ;
#3524=ORIENTED_EDGE ( 'NONE', *, *, #1540, .T. ) ;
#3527=CARTESIAN_POINT ( 'NONE',  ( 17.55913978494622896, -14.85518798308249266, -8.000000000000000000 ) ) ;
#3534=CARTESIAN_POINT ( 'NONE',  ( 17.74999999999999289, -15.01665741768121443, -4.000000000000000000 ) ) ;
#3539=LINE ( 'NONE', #1410, #4850 ) ;
#3540=ORIENTED_EDGE ( 'NONE', *, *, #4575, .T. ) ;
#3544=DIRECTION ( 'NONE',  ( 0.000000000000000000, 0.000000000000000000, -1.000000000000000000 ) ) ;
#3551=CIRCLE ( 'NONE', #1528, 25.00000000000000000 ) ;
#3554=ORIENTED_EDGE ( 'NONE', *, *, #352, .F. ) ;
#3579=ORIENTED_EDGE ( 'NONE', *, *, #3090, .F. ) ;
#3586=VERTEX_POINT ( 'NONE', #2417 ) ;
#3588=DIRECTION ( 'NONE',  ( -0.000000000000000000, -0.000000000000000000, 1.000000000000000000 ) ) ;
#3598=CARTESIAN_POINT ( 'NONE',  ( 4.999999999999914735, 24.49489742783179835, -8.000000000000000000 ) ) ;
#3624=CARTESIAN_POINT ( 'NONE',  ( 0.000000000000000000, 0.000000000000000000, -8.000000000000000000 ) ) ;
#3641=ORIENTED_EDGE ( 'NONE', *, *, #5258, .F. ) ;
#3650=EDGE_CURVE ( 'NONE', #4295, #4159, #5117, .T. ) ;
#3652=DIRECTION ( 'NONE',  ( 1.000000000000000000, 0.000000000000000000, 0.000000000000000000 ) ) ;
#3653=( NAMED_UNIT ( * ) PLANE_ANGLE_UNIT ( ) SI_UNIT ( $, .RADIAN. ) );
#3661=ADVANCED_FACE ( 'NONE', ( #2450 ), #3002, .T. ) ;
#3664=CARTESIAN_POINT ( 'NONE',  ( 23.48484848484848442, -8.570991287109677614, -8.000000000000000000 ) ) ;
#3685=DIRECTION ( 'NONE',  ( 1.000000000000000000, 0.000000000000000000, 0.000000000000000000 ) ) ;
#3692=DIRECTION ( 'NONE',  ( 1.000000000000000000, 0.000000000000000000, 0.000000000000000000 ) ) ;
#3695=CARTESIAN_POINT ( 'NONE',  ( 4.500000000000000888, 0.000000000000000000, 0.000000000000000000 ) ) ;
#3700=CARTESIAN_POINT ( 'NONE',  ( 0.000000000000000000, 0.000000000000000000, -8.000000000000000000 ) ) ;
#3708=CARTESIAN_POINT ( 'NONE',  ( 0.000000000000000000, 0.000000000000000000, 0.000000000000000000 ) ) ;
#3720=VECTOR ( 'NONE', #974, 1000.000000000000000 ) ;
#3729=ORIENTED_EDGE ( 'NONE', *, *, #3915, .T. ) ;
#3740=CIRCLE ( 'NONE', #4292, 25.00000000000000000 ) ;
#3747=CARTESIAN_POINT ( 'NONE',  ( -2.199999999999999289, 2.694222958124176020E-16, -3.100000000000000533 ) ) ;
#3752=EDGE_CURVE ( 'NONE', #5536, #4755, #1300, .T. ) ;
#3764=CARTESIAN_POINT ( 'NONE',  ( 0.000000000000000000, 0.000000000000000000, -8.000000000000000000 ) ) ;
#3767=ORIENTED_EDGE ( 'NONE', *, *, #4164, .F. ) ;
#3769=CARTESIAN_POINT ( 'NONE',  ( 0.000000000000000000, 0.000000000000000000, 0.000000000000000000 ) ) ;
#3776=CARTESIAN_POINT ( 'NONE',  ( 0.000000000000000000, 0.000000000000000000, -3.100000000000000533 ) ) ;
#3782=PLANE ( 'NONE',  #2255 ) ;
#3789=EDGE_LOOP ( 'NONE', ( #5226, #2050, #254, #5391 ) ) ;
#3792=CYLINDRICAL_SURFACE ( 'NONE', #3812, 0.2500000000000002220 ) ;
#3794=FACE_OUTER_BOUND ( 'NONE', #2467, .T. ) ;
#3800=ORIENTED_EDGE ( 'NONE', *, *, #5126, .T. ) ;
#3810=ORIENTED_EDGE ( 'NONE', *, *, #1368, .F. ) ;
#3812=AXIS2_PLACEMENT_3D ( 'NONE', #1979, #3365, #3307 ) ;
#3833=DIRECTION ( 'NONE',  ( -1.000000000000000000, 0.000000000000000000, 0.000000000000000000 ) ) ;
#3834=ORIENTED_EDGE ( 'NONE', *, *, #1274, .T. ) ;
#3835=DIRECTION ( 'NONE',  ( 1.000000000000000000, 0.000000000000000000, 0.000000000000000000 ) ) ;
#3842=FACE_OUTER_BOUND ( 'NONE', #3345, .T. ) ;
#3844=AXIS2_PLACEMENT_3D ( 'NONE', #5411, #2298, #1090 ) ;
#3849=VERTEX_POINT ( 'NONE', #284 ) ;
#3851=EDGE_CURVE ( 'NONE', #2920, #5392, #1731, .T. ) ;
#3860=ORIENTED_EDGE ( 'NONE', *, *, #559, .T. ) ;
#3888=CARTESIAN_POINT ( 'NONE',  ( 0.000000000000000000, 0.000000000000000000, -8.000000000000000000 ) ) ;
#3893=CARTESIAN_POINT ( 'NONE',  ( 23.24999999999999645, -8.485281374238580199, -8.000000000000000000 ) ) ;
#3898=UNCERTAINTY_MEASURE_WITH_UNIT (LENGTH_MEASURE( 1.000000000000000082E-05 ), #1554, 'distance_accuracy_value', 'NONE');
#3908=VECTOR ( 'NONE', #3111, 1000.000000000000000 ) ;
#3909=ADVANCED_FACE ( 'NONE', ( #370, #5637 ), #3452, .F. ) ;
#3913=AXIS2_PLACEMENT_3D ( 'NONE', #2169, #3433, #5648 ) ;
#3915=EDGE_CURVE ( 'NONE', #1283, #36, #1271, .T. ) ;
#3917=CARTESIAN_POINT ( 'NONE',  ( 0.000000000000000000, 0.000000000000000000, 0.000000000000000000 ) ) ;
#3919=AXIS2_PLACEMENT_3D ( 'NONE', #2936, #4688, #749 ) ;
#3926=ORIENTED_EDGE ( 'NONE', *, *, #5052, .F. ) ;
#3930=AXIS2_PLACEMENT_3D ( 'NONE', #1303, #3061, #4803 ) ;
#3935=EDGE_LOOP ( 'NONE', ( #5482, #3129, #485, #929 ) ) ;
#3941=CARTESIAN_POINT ( 'NONE',  ( 0.000000000000000000, 0.000000000000000000, -8.000000000000000000 ) ) ;
#3942=CARTESIAN_POINT ( 'NONE',  ( -2.149999999999998579, 2.632990618166807756E-16, -3.106350832689629637 ) ) ;
#3947=EDGE_CURVE ( 'NONE', #118, #4159, #1256, .T. ) ;
#3956=DIRECTION ( 'NONE',  ( 1.000000000000000000, 0.000000000000000000, 0.000000000000000000 ) ) ;
#3966=EDGE_CURVE ( 'NONE', #2746, #4295, #2242, .T. ) ;
#3971=LINE ( 'NONE', #1388, #4201 ) ;
#3973=EDGE_CURVE ( 'NONE', #4473, #4295, #2726, .T. ) ;
#3980=EDGE_CURVE ( 'NONE', #5536, #2168, #4651, .T. ) ;
#3983=EDGE_CURVE ( 'NONE', #726, #247, #3075, .T. ) ;
#3997=ADVANCED_FACE ( 'NONE', ( #28 ), #1813, .F. ) ;
#3999=DIRECTION ( 'NONE',  ( -0.000000000000000000, -0.000000000000000000, 1.000000000000000000 ) ) ;
#4001=VERTEX_POINT ( 'NONE', #3598 ) ;
#4008=ORIENTED_EDGE ( 'NONE', *, *, #679, .T. ) ;
#4025=ADVANCED_FACE ( 'NONE', ( #5384 ), #434, .F. ) ;
#4026=CIRCLE ( 'NONE', #1080, 5.000000000000000000 ) ;
#4028=FACE_OUTER_BOUND ( 'NONE', #2219, .T. ) ;
#4031=DIRECTION ( 'NONE',  ( -0.000000000000000000, -0.000000000000000000, 1.000000000000000000 ) ) ;
#4033=UNCERTAINTY_MEASURE_WITH_UNIT (LENGTH_MEASURE( 1.000000000000000082E-05 ), #314, 'distance_accuracy_value', 'NONE');
#4039=EDGE_LOOP ( 'NONE', ( #4942, #5464, #449, #4498 ) ) ;
#4056=ORIENTED_EDGE ( 'NONE', *, *, #1368, .T. ) ;
#4057=DIRECTION ( 'NONE',  ( 0.000000000000000000, 0.000000000000000000, -1.000000000000000000 ) ) ;
#4075=LINE ( 'NONE', #1507, #4304 ) ;
#4122=CARTESIAN_POINT ( 'NONE',  ( 22.99999999999999645, -8.485281374238580199, -8.000000000000000000 ) ) ;
#4131=CARTESIAN_POINT ( 'NONE',  ( -25.00000000000000000, 0.000000000000000000, 0.000000000000000000 ) ) ;
#4137=VERTEX_POINT ( 'NONE', #4917 ) ;
#4140=SURFACE_SIDE_STYLE ('',( #630 ) ) ;
#4146=ADVANCED_FACE ( 'NONE', ( #3056 ), #978, .T. ) ;
#4150=EDGE_LOOP ( 'NONE', ( #3834, #2013 ) ) ;
#4158=DIRECTION ( 'NONE',  ( -4.364351673553916694E-15, 1.000000000000000000, 0.000000000000000000 ) ) ;
#4159=VERTEX_POINT ( 'NONE', #3942 ) ;
#4164=EDGE_CURVE ( 'NONE', #4608, #4001, #401, .T. ) ;
#4176=EDGE_CURVE ( 'NONE', #3586, #964, #3167, .T. ) ;
#4178=DIRECTION ( 'NONE',  ( 0.000000000000000000, 0.000000000000000000, -1.000000000000000000 ) ) ;
#4201=VECTOR ( 'NONE', #2193, 1000.000000000000000 ) ;
#4212=DIRECTION ( 'NONE',  ( -0.000000000000000000, -0.000000000000000000, 1.000000000000000000 ) ) ;
#4227=PRODUCT ( 'outer cover 2', 'outer cover 2', '', ( #1833 ) ) ;
#4228=DIRECTION ( 'NONE',  ( -0.000000000000000000, -0.000000000000000000, 1.000000000000000000 ) ) ;
#4251=STYLED_ITEM ( 'NONE', ( #1518 ), #1651 ) ;
#4278=( GEOMETRIC_REPRESENTATION_CONTEXT ( 3 ) GLOBAL_UNCERTAINTY_ASSIGNED_CONTEXT ( ( #4033 ) ) GLOBAL_UNIT_ASSIGNED_CONTEXT ( ( #314, #5639, #2910 ) ) REPRESENTATION_CONTEXT ( 'NONE', 'WORKASPACE' ) );
#4292=AXIS2_PLACEMENT_3D ( 'NONE', #1525, #4604, #174 ) ;
#4295=VERTEX_POINT ( 'NONE', #4642 ) ;
#4304=VECTOR ( 'NONE', #161, 1000.000000000000000 ) ;
#4308=PRODUCT_DEFINITION_CONTEXT ( 'detailed design', #894, 'design' ) ;
#4309=CARTESIAN_POINT ( 'NONE',  ( 0.000000000000000000, 0.000000000000000000, -2.000000000000000000 ) ) ;
#4311=ORIENTED_EDGE ( 'NONE', *, *, #1423, .F. ) ;
#4327=CARTESIAN_POINT ( 'NONE',  ( 0.000000000000000000, 0.000000000000000000, -2.000000000000000000 ) ) ;
#4328=ORIENTED_EDGE ( 'NONE', *, *, #1995, .T. ) ;
#4344=EDGE_CURVE ( 'NONE', #1283, #5110, #3431, .T. ) ;
#4345=DIRECTION ( 'NONE',  ( -1.000000000000000000, 0.000000000000000000, 0.000000000000000000 ) ) ;
#4347=CARTESIAN_POINT ( 'NONE',  ( -2.199999999999999289, 2.694222958124176020E-16, -3.300000000000000266 ) ) ;
#4356=FACE_OUTER_BOUND ( 'NONE', #4039, .T. ) ;
#4367=DIRECTION ( 'NONE',  ( -4.364351673553916694E-15, 1.000000000000000000, 0.000000000000000000 ) ) ;
#4391=CARTESIAN_POINT ( 'NONE',  ( 0.000000000000000000, 0.000000000000000000, -8.000000000000000000 ) ) ;
#4406=CARTESIAN_POINT ( 'NONE',  ( 0.000000000000000000, 0.000000000000000000, -5.000000000000000000 ) ) ;
#4407=EDGE_CURVE ( 'NONE', #403, #4444, #3007, .T. ) ;
#4413=EDGE_CURVE ( 'NONE', #5110, #1556, #2607, .T. ) ;
#4419=FACE_OUTER_BOUND ( 'NONE', #2119, .T. ) ;
#4425=PLANE ( 'NONE',  #1790 ) ;
#4431=EDGE_CURVE ( 'NONE', #1283, #1326, #5305, .T. ) ;
#4433=CARTESIAN_POINT ( 'NONE',  ( 0.000000000000000000, 0.000000000000000000, 0.000000000000000000 ) ) ;
#4444=VERTEX_POINT ( 'NONE', #1280 ) ;
#4453=CARTESIAN_POINT ( 'NONE',  ( 25.00000000000000000, -3.061616997868383043E-15, -8.000000000000000000 ) ) ;
#4473=VERTEX_POINT ( 'NONE', #4781 ) ;
#4474=VECTOR ( 'NONE', #896, 1000.000000000000000 ) ;
#4480=EDGE_CURVE ( 'NONE', #3158, #964, #840, .T. ) ;
#4485=DIRECTION ( 'NONE',  ( -1.000000000000000000, 0.000000000000000000, 0.000000000000000000 ) ) ;
#4489=DIRECTION ( 'NONE',  ( 1.224646799147353207E-16, 1.000000000000000000, 0.000000000000000000 ) ) ;
#4497=ORIENTED_EDGE ( 'NONE', *, *, #4176, .T. ) ;
#4498=ORIENTED_EDGE ( 'NONE', *, *, #1866, .T. ) ;
#4509=ADVANCED_FACE ( 'NONE', ( #1874 ), #2248, .T. ) ;
#4521=CARTESIAN_POINT ( 'NONE',  ( 0.000000000000000000, 0.000000000000000000, -2.000000000000000000 ) ) ;
#4540=DIRECTION ( 'NONE',  ( -0.000000000000000000, -0.000000000000000000, 1.000000000000000000 ) ) ;
#4542=ORIENTED_EDGE ( 'NONE', *, *, #2529, .T. ) ;
#4547=DIRECTION ( 'NONE',  ( -0.000000000000000000, -0.000000000000000000, 1.000000000000000000 ) ) ;
#4548=ORIENTED_EDGE ( 'NONE', *, *, #5258, .T. ) ;
#4564=ORIENTED_EDGE ( 'NONE', *, *, #4344, .F. ) ;
#4565=EDGE_CURVE ( 'NONE', #1556, #5110, #2610, .T. ) ;
#4567=AXIS2_PLACEMENT_3D ( 'NONE', #804, #3397, #2125 ) ;
#4571=ORIENTED_EDGE ( 'NONE', *, *, #1423, .T. ) ;
#4572=CIRCLE ( 'NONE', #1363, 2.199999999999999289 ) ;
#4575=EDGE_CURVE ( 'NONE', #1283, #4764, #127, .T. ) ;
#4583=CARTESIAN_POINT ( 'NONE',  ( 17.74999999999999289, -15.01665741768121443, -8.000000000000000000 ) ) ;
#4591=EDGE_LOOP ( 'NONE', ( #2653, #3 ) ) ;
#4604=DIRECTION ( 'NONE',  ( -0.000000000000000000, -0.000000000000000000, 1.000000000000000000 ) ) ;
#4608=VERTEX_POINT ( 'NONE', #202 ) ;
#4633=AXIS2_PLACEMENT_3D ( 'NONE', #4309, #418, #447 ) ;
#4642=CARTESIAN_POINT ( 'NONE',  ( 2.149999999999998579, 0.000000000000000000, -3.106350832689629637 ) ) ;
#4651=CIRCLE ( 'NONE', #2175, 25.00000000000000000 ) ;
#4662=AXIS2_PLACEMENT_3D ( 'NONE', #4890, #3059, #864 ) ;
#4665=CARTESIAN_POINT ( 'NONE',  ( -5.000000000000076383, 22.44994432064363110, -5.000000000000000000 ) ) ;
#4674=CARTESIAN_POINT ( 'NONE',  ( 4.500000000000000888, 0.000000000000000000, 0.000000000000000000 ) ) ;
#4678=ORIENTED_EDGE ( 'NONE', *, *, #2950, .F. ) ;
#4682=DIRECTION ( 'NONE',  ( -1.000000000000000000, 0.000000000000000000, 0.000000000000000000 ) ) ;
#4688=DIRECTION ( 'NONE',  ( 0.000000000000000000, 0.000000000000000000, -1.000000000000000000 ) ) ;
#4695=DIRECTION ( 'NONE',  ( -1.000000000000000000, 0.000000000000000000, 0.000000000000000000 ) ) ;
#4716=ORIENTED_EDGE ( 'NONE', *, *, #4407, .F. ) ;
#4721=DIRECTION ( 'NONE',  ( -0.000000000000000000, -0.000000000000000000, 1.000000000000000000 ) ) ;
#4730=CARTESIAN_POINT ( 'NONE',  ( -5.000000000000085265, 24.49489742783176638, -8.000000000000000000 ) ) ;
#4734=AXIS2_PLACEMENT_3D ( 'NONE', #3893, #1654, #5618 ) ;
#4748=PLANE ( 'NONE',  #3099 ) ;
#4750=CIRCLE ( 'NONE', #68, 23.00000000000000000 ) ;
#4755=VERTEX_POINT ( 'NONE', #4730 ) ;
#4759=EDGE_CURVE ( 'NONE', #354, #3849, #3349, .T. ) ;
#4764=VERTEX_POINT ( 'NONE', #5624 ) ;
#4781=CARTESIAN_POINT ( 'NONE',  ( 2.199999999999999289, 0.000000000000000000, -3.100000000000000533 ) ) ;
#4784=ORIENTED_EDGE ( 'NONE', *, *, #4431, .F. ) ;
#4792=DIRECTION ( 'NONE',  ( 1.000000000000000000, 0.000000000000000000, 0.000000000000000000 ) ) ;
#4800=DIRECTION ( 'NONE',  ( -1.000000000000000000, 0.000000000000000000, 0.000000000000000000 ) ) ;
#4803=DIRECTION ( 'NONE',  ( 1.000000000000000000, 0.000000000000000000, 0.000000000000000000 ) ) ;
#4805=VECTOR ( 'NONE', #1706, 1000.000000000000000 ) ;
#4827=ADVANCED_FACE ( 'NONE', ( #878 ), #2637, .T. ) ;
#4837=DIRECTION ( 'NONE',  ( 1.000000000000000000, 0.000000000000000000, 0.000000000000000000 ) ) ;
#4839=CIRCLE ( 'NONE', #1989, 0.2500000000000002220 ) ;
#4850=VECTOR ( 'NONE', #4031, 1000.000000000000000 ) ;
#4858=PRODUCT_DEFINITION ( 'UNKNOWN', '', #298, #4308 ) ;
#4864=CYLINDRICAL_SURFACE ( 'NONE', #2366, 4.500000000000000888 ) ;
#4867=EDGE_CURVE ( 'NONE', #4764, #3158, #685, .T. ) ;
#4868=DIRECTION ( 'NONE',  ( -1.000000000000000000, 0.000000000000000000, 0.000000000000000000 ) ) ;
#4878=ORIENTED_EDGE ( 'NONE', *, *, #2535, .F. ) ;
#4886=DIRECTION ( 'NONE',  ( 1.000000000000000000, 0.000000000000000000, 0.000000000000000000 ) ) ;
#4890=CARTESIAN_POINT ( 'NONE',  ( 0.000000000000000000, 0.000000000000000000, -3.100000000000000533 ) ) ;
#4891=ORIENTED_EDGE ( 'NONE', *, *, #4344, .T. ) ;
#4894=CARTESIAN_POINT ( 'NONE',  ( -5.000000000000085265, 24.49489742783176638, -5.000000000000000000 ) ) ;
#4895=DIRECTION ( 'NONE',  ( -1.000000000000000000, 3.540989467475305966E-16, 0.000000000000000000 ) ) ;
#4902=EDGE_CURVE ( 'NONE', #1326, #726, #2674, .T. ) ;
#4917=CARTESIAN_POINT ( 'NONE',  ( 17.99999999999999289, -15.01665741768121443, -8.000000000000000000 ) ) ;
#4925=VECTOR ( 'NONE', #5609, 1000.000000000000000 ) ;
#4928=ORIENTED_EDGE ( 'NONE', *, *, #190, .F. ) ;
#4938=CARTESIAN_POINT ( 'NONE',  ( 4.999999999999914735, 24.49489742783179835, -5.000000000000000000 ) ) ;
#4942=ORIENTED_EDGE ( 'NONE', *, *, #5126, .F. ) ;
#4944=DIRECTION ( 'NONE',  ( -1.000000000000000000, 0.000000000000000000, 0.000000000000000000 ) ) ;
#4954=CYLINDRICAL_SURFACE ( 'NONE', #3449, 5.000000000000000000 ) ;
#4968=LINE ( 'NONE', #2784, #1696 ) ;
#4970=ORIENTED_EDGE ( 'NONE', *, *, #3090, .T. ) ;
#4975=ORIENTED_EDGE ( 'NONE', *, *, #352, .T. ) ;
#4984=LINE ( 'NONE', #2371, #1339 ) ;
#4986=CARTESIAN_POINT ( 'NONE',  ( 17.99999999999999289, -17.34935157289748631, -4.000000000000000000 ) ) ;
#4992=VERTEX_POINT ( 'NONE', #480 ) ;
#5009=VERTEX_POINT ( 'NONE', #82 ) ;
#5014=VECTOR ( 'NONE', #2500, 1000.000000000000000 ) ;
#5017=ADVANCED_FACE ( 'NONE', ( #1810 ), #2187, .T. ) ;
#5028=CARTESIAN_POINT ( 'NONE',  ( 23.00000000000000000, -2.816687638038912352E-15, -2.000000000000000000 ) ) ;
#5030=( NAMED_UNIT ( * ) SI_UNIT ( $, .STERADIAN. ) SOLID_ANGLE_UNIT ( ) );
#5033=AXIS2_PLACEMENT_3D ( 'NONE', #3131, #1745, #4367 ) ;
#5035=DIRECTION ( 'NONE',  ( -1.000000000000000000, 0.000000000000000000, 0.000000000000000000 ) ) ;
#5052=EDGE_CURVE ( 'NONE', #4608, #1240, #2269, .T. ) ;
#5054=ORIENTED_EDGE ( 'NONE', *, *, #1982, .F. ) ;
#5063=ADVANCED_FACE ( 'NONE', ( #4028 ), #5212, .F. ) ;
#5065=VERTEX_POINT ( 'NONE', #5406 ) ;
#5074=ORIENTED_EDGE ( 'NONE', *, *, #429, .T. ) ;
#5079=EDGE_CURVE ( 'NONE', #4137, #1719, #976, .T. ) ;
#5107=ORIENTED_EDGE ( 'NONE', *, *, #1274, .F. ) ;
#5108=CARTESIAN_POINT ( 'NONE',  ( -5.000000000000000000, 4.999999999999978684, -8.000000000000000000 ) ) ;
#5110=VERTEX_POINT ( 'NONE', #5028 ) ;
#5117=CIRCLE ( 'NONE', #706, 2.149999999999998579 ) ;
#5126=EDGE_CURVE ( 'NONE', #2224, #442, #4968, .T. ) ;
#5143=ORIENTED_EDGE ( 'NONE', *, *, #4, .F. ) ;
#5146=EDGE_CURVE ( 'NONE', #1251, #5065, #43, .T. ) ;
#5154=CARTESIAN_POINT ( 'NONE',  ( -5.000000000000085265, 24.49489742783176638, -8.000000000000000000 ) ) ;
#5196=CIRCLE ( 'NONE', #1243, 2.149999999999998579 ) ;
#5205=VECTOR ( 'NONE', #1385, 1000.000000000000000 ) ;
#5206=DIRECTION ( 'NONE',  ( -0.000000000000000000, -0.000000000000000000, 1.000000000000000000 ) ) ;
#5207=AXIS2_PLACEMENT_3D ( 'NONE', #1823, #5279, #1335 ) ;
#5212=CYLINDRICAL_SURFACE ( 'NONE', #1604, 2.149999999999998579 ) ;
#5213=DIRECTION ( 'NONE',  ( 1.000000000000000000, 0.000000000000000000, 0.000000000000000000 ) ) ;
#5217=LINE ( 'NONE', #2478, #968 ) ;
#5226=ORIENTED_EDGE ( 'NONE', *, *, #2017, .T. ) ;
#5233=ORIENTED_EDGE ( 'NONE', *, *, #4902, .T. ) ;
#5235=EDGE_CURVE ( 'NONE', #1305, #2861, #629, .T. ) ;
#5246=EDGE_LOOP ( 'NONE', ( #1579, #4548, #2479, #2502 ) ) ;
#5250=ORIENTED_EDGE ( 'NONE', *, *, #2535, .T. ) ;
#5258=EDGE_CURVE ( 'NONE', #4992, #2140, #2709, .T. ) ;
#5266=ADVANCED_FACE ( 'NONE', ( #1009, #637 ), #3228, .F. ) ;
#5272=CARTESIAN_POINT ( 'NONE',  ( 5.000000000000000000, 5.000000000000022204, -8.000000000000000000 ) ) ;
#5273=DIRECTION ( 'NONE',  ( -0.000000000000000000, -0.000000000000000000, -1.000000000000000000 ) ) ;
#5274=VECTOR ( 'NONE', #2568, 1000.000000000000000 ) ;
#5278=EDGE_LOOP ( 'NONE', ( #3810, #5054 ) ) ;
#5279=DIRECTION ( 'NONE',  ( -0.000000000000000000, -0.000000000000000000, 1.000000000000000000 ) ) ;
#5289=CARTESIAN_POINT ( 'NONE',  ( 0.000000000000000000, 0.000000000000000000, -8.000000000000000000 ) ) ;
#5298=CARTESIAN_POINT ( 'NONE',  ( 23.00000000000000000, -8.144275775193202933E-15, -4.000000000000000000 ) ) ;
#5300=AXIS2_PLACEMENT_3D ( 'NONE', #2419, #2799, #1013 ) ;
#5305=LINE ( 'NONE', #5616, #4805 ) ;
#5323=DIRECTION ( 'NONE',  ( -0.000000000000000000, -0.000000000000000000, 1.000000000000000000 ) ) ;
#5328=ADVANCED_FACE ( 'NONE', ( #1143 ), #3792, .T. ) ;
#5330=DIRECTION ( 'NONE',  ( 1.000000000000000000, 0.000000000000000000, 0.000000000000000000 ) ) ;
#5333=ORIENTED_EDGE ( 'NONE', *, *, #4407, .T. ) ;
#5367=ORIENTED_EDGE ( 'NONE', *, *, #412, .F. ) ;
#5378=FACE_OUTER_BOUND ( 'NONE', #3935, .T. ) ;
#5382=CIRCLE ( 'NONE', #2992, 0.2500000000000002220 ) ;
#5384=FACE_OUTER_BOUND ( 'NONE', #1440, .T. ) ;
#5387=VECTOR ( 'NONE', #285, 1000.000000000000000 ) ;
#5391=ORIENTED_EDGE ( 'NONE', *, *, #2700, .F. ) ;
#5392=VERTEX_POINT ( 'NONE', #2929 ) ;
#5406=CARTESIAN_POINT ( 'NONE',  ( 17.55913978494622896, -14.85518798308249266, -8.000000000000000000 ) ) ;
#5411=CARTESIAN_POINT ( 'NONE',  ( 0.000000000000000000, 0.000000000000000000, -2.000000000000000000 ) ) ;
#5415=DIRECTION ( 'NONE',  ( -1.000000000000000000, 0.000000000000000000, 0.000000000000000000 ) ) ;
#5428=ADVANCED_FACE ( 'NONE', ( #1577 ), #1605, .T. ) ;
#5450=ORIENTED_EDGE ( 'NONE', *, *, #2896, .T. ) ;
#5452=DIRECTION ( 'NONE',  ( 1.000000000000000000, 0.000000000000000000, 0.000000000000000000 ) ) ;
#5456=AXIS2_PLACEMENT_3D ( 'NONE', #1781, #545, #3170 ) ;
#5457=EDGE_LOOP ( 'NONE', ( #325, #5074, #4008, #3767, #2911, #1146 ) ) ;
#5460=DIRECTION ( 'NONE',  ( -3.540989467475305966E-16, -1.000000000000000000, -0.000000000000000000 ) ) ;
#5461=SURFACE_STYLE_USAGE ( .BOTH. , #4140 ) ;
#5464=ORIENTED_EDGE ( 'NONE', *, *, #2300, .F. ) ;
#5468=AXIS2_PLACEMENT_3D ( 'NONE', #3776, #5474, #3347 ) ;
#5473=FACE_OUTER_BOUND ( 'NONE', #2898, .T. ) ;
#5474=DIRECTION ( 'NONE',  ( -0.000000000000000000, -0.000000000000000000, 1.000000000000000000 ) ) ;
#5482=ORIENTED_EDGE ( 'NONE', *, *, #2032, .T. ) ;
#5491=CIRCLE ( 'NONE', #4662, 2.199999999999999289 ) ;
#5516=EDGE_LOOP ( 'NONE', ( #3926, #1155, #232, #1221, #5678, #3332, #2435, #5143 ) ) ;
#5527=EDGE_CURVE ( 'NONE', #403, #2920, #1509, .T. ) ;
#5533=ADVANCED_FACE ( 'NONE', ( #924 ), #2679, .F. ) ;
#5535=CARTESIAN_POINT ( 'NONE',  ( 0.000000000000000000, 0.000000000000000000, -8.000000000000000000 ) ) ;
#5536=VERTEX_POINT ( 'NONE', #4894 ) ;
#5537=DIRECTION ( 'NONE',  ( 0.000000000000000000, 0.000000000000000000, -1.000000000000000000 ) ) ;
#5554=VECTOR ( 'NONE', #5460, 1000.000000000000000 ) ;
#5587=EDGE_LOOP ( 'NONE', ( #2184, #1531 ) ) ;
#5594=CYLINDRICAL_SURFACE ( 'NONE', #4734, 0.2500000000000002220 ) ;
#5609=DIRECTION ( 'NONE',  ( 0.000000000000000000, 0.000000000000000000, -1.000000000000000000 ) ) ;
#5610=LINE ( 'NONE', #1671, #5387 ) ;
#5613=CARTESIAN_POINT ( 'NONE',  ( 0.000000000000000000, 0.000000000000000000, -3.106350832689629637 ) ) ;
#5616=CARTESIAN_POINT ( 'NONE',  ( 23.00000000000000000, -2.168404344971008868E-16, 16.41957833606399930 ) ) ;
#5618=DIRECTION ( 'NONE',  ( -1.000000000000000000, 0.000000000000000000, 0.000000000000000000 ) ) ;
#5619=ORIENTED_EDGE ( 'NONE', *, *, #2032, .F. ) ;
#5624=CARTESIAN_POINT ( 'NONE',  ( 17.55913978494622896, -14.85518798308249266, -4.000000000000000000 ) ) ;
#5637=FACE_BOUND ( 'NONE', #5278, .T. ) ;
#5639=( NAMED_UNIT ( * ) PLANE_ANGLE_UNIT ( ) SI_UNIT ( $, .RADIAN. ) );
#5641=DIRECTION ( 'NONE',  ( 0.000000000000000000, 0.000000000000000000, -1.000000000000000000 ) ) ;
#5642=LINE ( 'NONE', #2565, #3720 ) ;
#5644=AXIS2_PLACEMENT_3D ( 'NONE', #4391, #2204, #3956 ) ;
#5648=DIRECTION ( 'NONE',  ( 1.000000000000000000, 0.000000000000000000, 0.000000000000000000 ) ) ;
#5649=ORIENTED_EDGE ( 'NONE', *, *, #2544, .F. ) ;
#5655=MECHANICAL_DESIGN_GEOMETRIC_PRESENTATION_REPRESENTATION('',(#3266),#4278);
#5671=DIRECTION ( 'NONE',  ( 1.000000000000000000, 0.000000000000000000, 0.000000000000000000 ) ) ;
#5675=ADVANCED_FACE ( 'NONE', ( #1121 ), #3085, .T. ) ;
#5678=ORIENTED_EDGE ( 'NONE', *, *, #3752, .T. ) ;
#5703=COLOUR_RGB('Light Blue',0.38,0.62,0.78);
#5704=FILL_AREA_STYLE_COLOUR('',#5703);
#5705=FILL_AREA_STYLE('',(#5704));
#5706=SURFACE_STYLE_FILL_AREA(#5705);
#5707=SURFACE_SIDE_STYLE('',(#5706));
#5708=SURFACE_STYLE_USAGE(.BOTH.,#5707);
#5709=PRESENTATION_STYLE_ASSIGNMENT((#5708));
ENDSEC;
END-ISO-10303-21;
